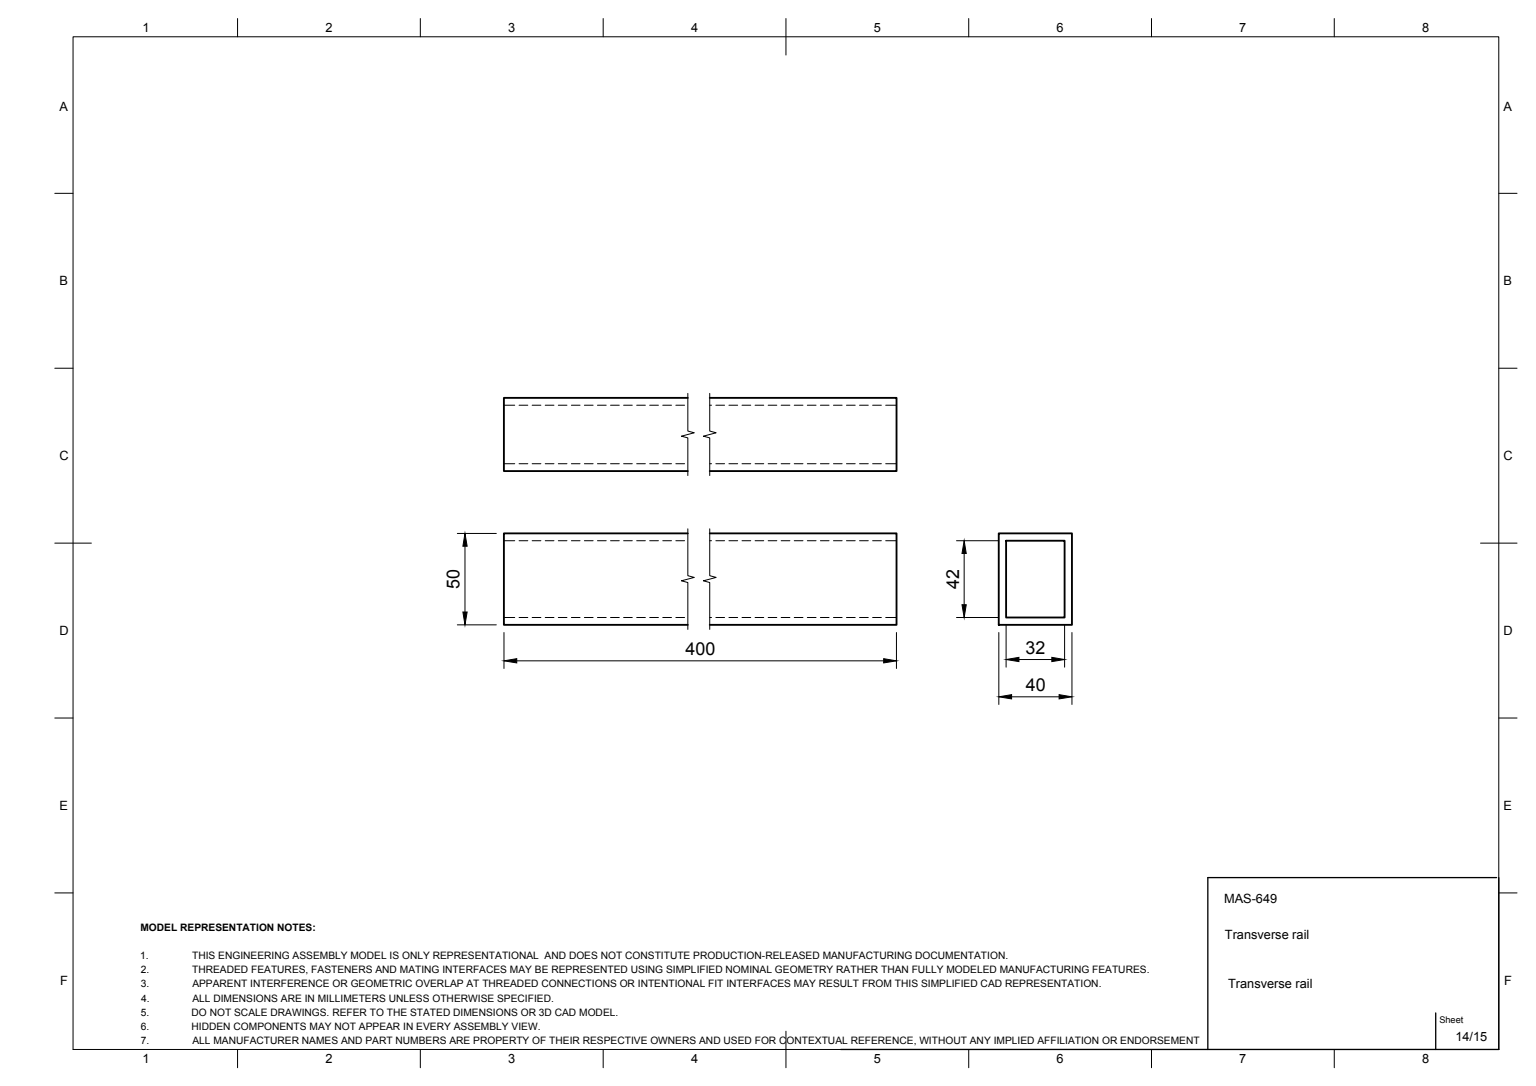
ISO-10303-21;
HEADER;
/* Generated by software containing ST-Developer
 * from STEP Tools, Inc. (www.steptools.com) 
 */

FILE_DESCRIPTION(
/* description */ ('Independent equipment support assembly with bolted 600 x 500 mm welde
d perimeter frame, four adjustable legs and swivel feet. Nominal overa
ll height 518 mm. No load rating assigned.'),
/* implementation_level */ '2;1');

FILE_NAME(
/* name */ 'Transverse rail.step',
/* time_stamp */ '2026-11-07T17:30:39-08:00',
/* author */ (''),
/* organization */ (''),
/* preprocessor_version */ 'ST-DEVELOPER v20.2',
/* originating_system */ 'Autodesk Translation Framework v15.17.0.0',
/* authorisation */ '');

FILE_SCHEMA (('AUTOMOTIVE_DESIGN { 1 0 10303 214 3 1 1 }'));
ENDSEC;

DATA;
#10=MECHANICAL_DESIGN_GEOMETRIC_PRESENTATION_REPRESENTATION('',(#2209),#63755);
#2177=SHAPE_REPRESENTATION_RELATIONSHIP('SRR','None',#63861,#2193);
#2193=ADVANCED_BREP_SHAPE_REPRESENTATION('',(#2225),#63739);
#2209=STYLED_ITEM('',(#63958),#2225);
#2225=MANIFOLD_SOLID_BREP('Body1',#14310);
#2242=FACE_BOUND('',#3084,.T.);
#2243=FACE_BOUND('',#3086,.T.);
#2313=FACE_OUTER_BOUND('',#3075,.T.);
#2314=FACE_OUTER_BOUND('',#3076,.T.);
#2315=FACE_OUTER_BOUND('',#3077,.T.);
#2316=FACE_OUTER_BOUND('',#3078,.T.);
#2317=FACE_OUTER_BOUND('',#3079,.T.);
#2318=FACE_OUTER_BOUND('',#3080,.T.);
#2319=FACE_OUTER_BOUND('',#3081,.T.);
#2320=FACE_OUTER_BOUND('',#3082,.T.);
#2321=FACE_OUTER_BOUND('',#3083,.T.);
#2322=FACE_OUTER_BOUND('',#3085,.T.);
#3075=EDGE_LOOP('',(#9175,#9176,#9177,#9178));
#3076=EDGE_LOOP('',(#9179,#9180,#9181,#9182));
#3077=EDGE_LOOP('',(#9183,#9184,#9185,#9186));
#3078=EDGE_LOOP('',(#9187,#9188,#9189,#9190));
#3079=EDGE_LOOP('',(#9191,#9192,#9193,#9194));
#3080=EDGE_LOOP('',(#9195,#9196,#9197,#9198));
#3081=EDGE_LOOP('',(#9199,#9200,#9201,#9202));
#3082=EDGE_LOOP('',(#9203,#9204,#9205,#9206));
#3083=EDGE_LOOP('',(#9207,#9208,#9209,#9210));
#3084=EDGE_LOOP('',(#9211,#9212,#9213,#9214));
#3085=EDGE_LOOP('',(#9215,#9216,#9217,#9218));
#3086=EDGE_LOOP('',(#9219,#9220,#9221,#9222));
#3910=LINE('',#18434,#4746);
#3911=LINE('',#18436,#4747);
#3912=LINE('',#18438,#4748);
#3913=LINE('',#18439,#4749);
#3914=LINE('',#18442,#4750);
#3915=LINE('',#18444,#4751);
#3916=LINE('',#18445,#4752);
#3917=LINE('',#18448,#4753);
#3918=LINE('',#18450,#4754);
#3919=LINE('',#18451,#4755);
#3920=LINE('',#18453,#4756);
#3921=LINE('',#18454,#4757);
#3922=LINE('',#18458,#4758);
#3923=LINE('',#18460,#4759);
#3924=LINE('',#18462,#4760);
#3925=LINE('',#18463,#4761);
#3926=LINE('',#18466,#4762);
#3927=LINE('',#18468,#4763);
#3928=LINE('',#18469,#4764);
#3929=LINE('',#18472,#4765);
#3930=LINE('',#18474,#4766);
#3931=LINE('',#18475,#4767);
#3932=LINE('',#18477,#4768);
#3933=LINE('',#18478,#4769);
#4746=VECTOR('',#15569,10.);
#4747=VECTOR('',#15570,10.);
#4748=VECTOR('',#15571,10.);
#4749=VECTOR('',#15572,10.);
#4750=VECTOR('',#15575,10.);
#4751=VECTOR('',#15576,10.);
#4752=VECTOR('',#15577,10.);
#4753=VECTOR('',#15580,10.);
#4754=VECTOR('',#15581,10.);
#4755=VECTOR('',#15582,10.);
#4756=VECTOR('',#15585,10.);
#4757=VECTOR('',#15586,10.);
#4758=VECTOR('',#15589,10.);
#4759=VECTOR('',#15590,10.);
#4760=VECTOR('',#15591,10.);
#4761=VECTOR('',#15592,10.);
#4762=VECTOR('',#15595,10.);
#4763=VECTOR('',#15596,10.);
#4764=VECTOR('',#15597,10.);
#4765=VECTOR('',#15600,10.);
#4766=VECTOR('',#15601,10.);
#4767=VECTOR('',#15602,10.);
#4768=VECTOR('',#15605,10.);
#4769=VECTOR('',#15606,10.);
#5574=VERTEX_POINT('',#18432);
#5575=VERTEX_POINT('',#18433);
#5576=VERTEX_POINT('',#18435);
#5577=VERTEX_POINT('',#18437);
#5578=VERTEX_POINT('',#18441);
#5579=VERTEX_POINT('',#18443);
#5580=VERTEX_POINT('',#18447);
#5581=VERTEX_POINT('',#18449);
#5582=VERTEX_POINT('',#18456);
#5583=VERTEX_POINT('',#18457);
#5584=VERTEX_POINT('',#18459);
#5585=VERTEX_POINT('',#18461);
#5586=VERTEX_POINT('',#18465);
#5587=VERTEX_POINT('',#18467);
#5588=VERTEX_POINT('',#18471);
#5589=VERTEX_POINT('',#18473);
#7010=EDGE_CURVE('',#5574,#5575,#3910,.T.);
#7011=EDGE_CURVE('',#5575,#5576,#3911,.T.);
#7012=EDGE_CURVE('',#5577,#5576,#3912,.T.);
#7013=EDGE_CURVE('',#5574,#5577,#3913,.T.);
#7014=EDGE_CURVE('',#5578,#5574,#3914,.T.);
#7015=EDGE_CURVE('',#5579,#5577,#3915,.T.);
#7016=EDGE_CURVE('',#5578,#5579,#3916,.T.);
#7017=EDGE_CURVE('',#5580,#5578,#3917,.T.);
#7018=EDGE_CURVE('',#5581,#5579,#3918,.T.);
#7019=EDGE_CURVE('',#5580,#5581,#3919,.T.);
#7020=EDGE_CURVE('',#5575,#5580,#3920,.T.);
#7021=EDGE_CURVE('',#5576,#5581,#3921,.T.);
#7022=EDGE_CURVE('',#5582,#5583,#3922,.T.);
#7023=EDGE_CURVE('',#5583,#5584,#3923,.T.);
#7024=EDGE_CURVE('',#5585,#5584,#3924,.T.);
#7025=EDGE_CURVE('',#5582,#5585,#3925,.T.);
#7026=EDGE_CURVE('',#5586,#5582,#3926,.T.);
#7027=EDGE_CURVE('',#5587,#5585,#3927,.T.);
#7028=EDGE_CURVE('',#5586,#5587,#3928,.T.);
#7029=EDGE_CURVE('',#5588,#5586,#3929,.T.);
#7030=EDGE_CURVE('',#5589,#5587,#3930,.T.);
#7031=EDGE_CURVE('',#5588,#5589,#3931,.T.);
#7032=EDGE_CURVE('',#5583,#5588,#3932,.T.);
#7033=EDGE_CURVE('',#5584,#5589,#3933,.T.);
#9175=ORIENTED_EDGE('',*,*,#7010,.T.);
#9176=ORIENTED_EDGE('',*,*,#7011,.T.);
#9177=ORIENTED_EDGE('',*,*,#7012,.F.);
#9178=ORIENTED_EDGE('',*,*,#7013,.F.);
#9179=ORIENTED_EDGE('',*,*,#7014,.T.);
#9180=ORIENTED_EDGE('',*,*,#7013,.T.);
#9181=ORIENTED_EDGE('',*,*,#7015,.F.);
#9182=ORIENTED_EDGE('',*,*,#7016,.F.);
#9183=ORIENTED_EDGE('',*,*,#7017,.T.);
#9184=ORIENTED_EDGE('',*,*,#7016,.T.);
#9185=ORIENTED_EDGE('',*,*,#7018,.F.);
#9186=ORIENTED_EDGE('',*,*,#7019,.F.);
#9187=ORIENTED_EDGE('',*,*,#7020,.T.);
#9188=ORIENTED_EDGE('',*,*,#7019,.T.);
#9189=ORIENTED_EDGE('',*,*,#7021,.F.);
#9190=ORIENTED_EDGE('',*,*,#7011,.F.);
#9191=ORIENTED_EDGE('',*,*,#7022,.T.);
#9192=ORIENTED_EDGE('',*,*,#7023,.T.);
#9193=ORIENTED_EDGE('',*,*,#7024,.F.);
#9194=ORIENTED_EDGE('',*,*,#7025,.F.);
#9195=ORIENTED_EDGE('',*,*,#7026,.T.);
#9196=ORIENTED_EDGE('',*,*,#7025,.T.);
#9197=ORIENTED_EDGE('',*,*,#7027,.F.);
#9198=ORIENTED_EDGE('',*,*,#7028,.F.);
#9199=ORIENTED_EDGE('',*,*,#7029,.T.);
#9200=ORIENTED_EDGE('',*,*,#7028,.T.);
#9201=ORIENTED_EDGE('',*,*,#7030,.F.);
#9202=ORIENTED_EDGE('',*,*,#7031,.F.);
#9203=ORIENTED_EDGE('',*,*,#7032,.T.);
#9204=ORIENTED_EDGE('',*,*,#7031,.T.);
#9205=ORIENTED_EDGE('',*,*,#7033,.F.);
#9206=ORIENTED_EDGE('',*,*,#7023,.F.);
#9207=ORIENTED_EDGE('',*,*,#7033,.T.);
#9208=ORIENTED_EDGE('',*,*,#7030,.T.);
#9209=ORIENTED_EDGE('',*,*,#7027,.T.);
#9210=ORIENTED_EDGE('',*,*,#7024,.T.);
#9211=ORIENTED_EDGE('',*,*,#7021,.T.);
#9212=ORIENTED_EDGE('',*,*,#7018,.T.);
#9213=ORIENTED_EDGE('',*,*,#7015,.T.);
#9214=ORIENTED_EDGE('',*,*,#7012,.T.);
#9215=ORIENTED_EDGE('',*,*,#7032,.F.);
#9216=ORIENTED_EDGE('',*,*,#7022,.F.);
#9217=ORIENTED_EDGE('',*,*,#7026,.F.);
#9218=ORIENTED_EDGE('',*,*,#7029,.F.);
#9219=ORIENTED_EDGE('',*,*,#7020,.F.);
#9220=ORIENTED_EDGE('',*,*,#7010,.F.);
#9221=ORIENTED_EDGE('',*,*,#7014,.F.);
#9222=ORIENTED_EDGE('',*,*,#7017,.F.);
#13419=PLANE('',#14516);
#13420=PLANE('',#14517);
#13421=PLANE('',#14518);
#13422=PLANE('',#14519);
#13423=PLANE('',#14520);
#13424=PLANE('',#14521);
#13425=PLANE('',#14522);
#13426=PLANE('',#14523);
#13427=PLANE('',#14524);
#13428=PLANE('',#14525);
#13559=ADVANCED_FACE('',(#2313),#13419,.T.);
#13560=ADVANCED_FACE('',(#2314),#13420,.T.);
#13561=ADVANCED_FACE('',(#2315),#13421,.T.);
#13562=ADVANCED_FACE('',(#2316),#13422,.T.);
#13563=ADVANCED_FACE('',(#2317),#13423,.T.);
#13564=ADVANCED_FACE('',(#2318),#13424,.T.);
#13565=ADVANCED_FACE('',(#2319),#13425,.T.);
#13566=ADVANCED_FACE('',(#2320),#13426,.T.);
#13567=ADVANCED_FACE('',(#2321,#2242),#13427,.T.);
#13568=ADVANCED_FACE('',(#2322,#2243),#13428,.F.);
#14310=CLOSED_SHELL('',(#13559,#13560,#13561,#13562,#13563,#13564,#13565,
#13566,#13567,#13568));
#14515=AXIS2_PLACEMENT_3D('',#18430,#15565,#15566);
#14516=AXIS2_PLACEMENT_3D('',#18431,#15567,#15568);
#14517=AXIS2_PLACEMENT_3D('',#18440,#15573,#15574);
#14518=AXIS2_PLACEMENT_3D('',#18446,#15578,#15579);
#14519=AXIS2_PLACEMENT_3D('',#18452,#15583,#15584);
#14520=AXIS2_PLACEMENT_3D('',#18455,#15587,#15588);
#14521=AXIS2_PLACEMENT_3D('',#18464,#15593,#15594);
#14522=AXIS2_PLACEMENT_3D('',#18470,#15598,#15599);
#14523=AXIS2_PLACEMENT_3D('',#18476,#15603,#15604);
#14524=AXIS2_PLACEMENT_3D('',#18479,#15607,#15608);
#14525=AXIS2_PLACEMENT_3D('',#18480,#15609,#15610);
#15565=DIRECTION('axis',(0.,0.,1.));
#15566=DIRECTION('refdir',(1.,0.,0.));
#15567=DIRECTION('center_axis',(0.,1.,0.));
#15568=DIRECTION('ref_axis',(-1.,0.,0.));
#15569=DIRECTION('',(-1.,0.,0.));
#15570=DIRECTION('',(0.,0.,1.));
#15571=DIRECTION('',(-1.,0.,0.));
#15572=DIRECTION('',(0.,0.,1.));
#15573=DIRECTION('center_axis',(-1.,0.,0.));
#15574=DIRECTION('ref_axis',(0.,-1.,0.));
#15575=DIRECTION('',(0.,-1.,0.));
#15576=DIRECTION('',(0.,-1.,0.));
#15577=DIRECTION('',(0.,0.,1.));
#15578=DIRECTION('center_axis',(0.,-1.,0.));
#15579=DIRECTION('ref_axis',(1.,0.,0.));
#15580=DIRECTION('',(1.,0.,0.));
#15581=DIRECTION('',(1.,0.,0.));
#15582=DIRECTION('',(0.,0.,1.));
#15583=DIRECTION('center_axis',(1.,0.,0.));
#15584=DIRECTION('ref_axis',(0.,1.,0.));
#15585=DIRECTION('',(0.,1.,0.));
#15586=DIRECTION('',(0.,1.,0.));
#15587=DIRECTION('center_axis',(0.,1.,0.));
#15588=DIRECTION('ref_axis',(-1.,0.,0.));
#15589=DIRECTION('',(-1.,0.,0.));
#15590=DIRECTION('',(0.,0.,1.));
#15591=DIRECTION('',(-1.,0.,0.));
#15592=DIRECTION('',(0.,0.,1.));
#15593=DIRECTION('center_axis',(1.,0.,0.));
#15594=DIRECTION('ref_axis',(0.,1.,0.));
#15595=DIRECTION('',(0.,1.,0.));
#15596=DIRECTION('',(0.,1.,0.));
#15597=DIRECTION('',(0.,0.,1.));
#15598=DIRECTION('center_axis',(0.,-1.,0.));
#15599=DIRECTION('ref_axis',(1.,0.,0.));
#15600=DIRECTION('',(1.,0.,0.));
#15601=DIRECTION('',(1.,0.,0.));
#15602=DIRECTION('',(0.,0.,1.));
#15603=DIRECTION('center_axis',(-1.,0.,0.));
#15604=DIRECTION('ref_axis',(0.,-1.,0.));
#15605=DIRECTION('',(0.,-1.,0.));
#15606=DIRECTION('',(0.,-1.,0.));
#15607=DIRECTION('center_axis',(0.,0.,1.));
#15608=DIRECTION('ref_axis',(1.,0.,0.));
#15609=DIRECTION('center_axis',(0.,0.,1.));
#15610=DIRECTION('ref_axis',(1.,0.,0.));
#18430=CARTESIAN_POINT('',(0.,0.,0.));
#18431=CARTESIAN_POINT('Origin',(16.,-21.,0.));
#18432=CARTESIAN_POINT('',(16.,-21.,0.));
#18433=CARTESIAN_POINT('',(-16.,-21.,0.));
#18434=CARTESIAN_POINT('',(-16.,-21.,0.));
#18435=CARTESIAN_POINT('',(-16.,-21.,400.));
#18436=CARTESIAN_POINT('',(-16.,-21.,0.));
#18437=CARTESIAN_POINT('',(16.,-21.,400.));
#18438=CARTESIAN_POINT('',(-16.,-21.,400.));
#18439=CARTESIAN_POINT('',(16.,-21.,0.));
#18440=CARTESIAN_POINT('Origin',(16.,21.,0.));
#18441=CARTESIAN_POINT('',(16.,21.,0.));
#18442=CARTESIAN_POINT('',(16.,-21.,0.));
#18443=CARTESIAN_POINT('',(16.,21.,400.));
#18444=CARTESIAN_POINT('',(16.,-21.,400.));
#18445=CARTESIAN_POINT('',(16.,21.,0.));
#18446=CARTESIAN_POINT('Origin',(-16.,21.,0.));
#18447=CARTESIAN_POINT('',(-16.,21.,0.));
#18448=CARTESIAN_POINT('',(16.,21.,0.));
#18449=CARTESIAN_POINT('',(-16.,21.,400.));
#18450=CARTESIAN_POINT('',(16.,21.,400.));
#18451=CARTESIAN_POINT('',(-16.,21.,0.));
#18452=CARTESIAN_POINT('Origin',(-16.,-21.,0.));
#18453=CARTESIAN_POINT('',(-16.,21.,0.));
#18454=CARTESIAN_POINT('',(-16.,21.,400.));
#18455=CARTESIAN_POINT('Origin',(20.,25.,0.));
#18456=CARTESIAN_POINT('',(20.,25.,0.));
#18457=CARTESIAN_POINT('',(-20.,25.,0.));
#18458=CARTESIAN_POINT('',(20.,25.,0.));
#18459=CARTESIAN_POINT('',(-20.,25.,400.));
#18460=CARTESIAN_POINT('',(-20.,25.,0.));
#18461=CARTESIAN_POINT('',(20.,25.,400.));
#18462=CARTESIAN_POINT('',(20.,25.,400.));
#18463=CARTESIAN_POINT('',(20.,25.,0.));
#18464=CARTESIAN_POINT('Origin',(20.,-25.,0.));
#18465=CARTESIAN_POINT('',(20.,-25.,0.));
#18466=CARTESIAN_POINT('',(20.,-25.,0.));
#18467=CARTESIAN_POINT('',(20.,-25.,400.));
#18468=CARTESIAN_POINT('',(20.,-25.,400.));
#18469=CARTESIAN_POINT('',(20.,-25.,0.));
#18470=CARTESIAN_POINT('Origin',(-20.,-25.,0.));
#18471=CARTESIAN_POINT('',(-20.,-25.,0.));
#18472=CARTESIAN_POINT('',(-20.,-25.,0.));
#18473=CARTESIAN_POINT('',(-20.,-25.,400.));
#18474=CARTESIAN_POINT('',(-20.,-25.,400.));
#18475=CARTESIAN_POINT('',(-20.,-25.,0.));
#18476=CARTESIAN_POINT('Origin',(-20.,25.,0.));
#18477=CARTESIAN_POINT('',(-20.,25.,0.));
#18478=CARTESIAN_POINT('',(-20.,25.,400.));
#18479=CARTESIAN_POINT('Origin',(0.,0.,400.));
#18480=CARTESIAN_POINT('Origin',(0.,0.,0.));
#63719=UNCERTAINTY_MEASURE_WITH_UNIT(LENGTH_MEASURE(0.01),#63756,
'DISTANCE_ACCURACY_VALUE',
'Maximum model space distance between geometric entities at asserted c
onnectivities');
#63735=UNCERTAINTY_MEASURE_WITH_UNIT(LENGTH_MEASURE(0.01),#63756,
'DISTANCE_ACCURACY_VALUE',
'Maximum model space distance between geometric entities at asserted c
onnectivities');
#63739=(
GEOMETRIC_REPRESENTATION_CONTEXT(3)
GLOBAL_UNCERTAINTY_ASSIGNED_CONTEXT((#63719))
GLOBAL_UNIT_ASSIGNED_CONTEXT((#63756,#63758,#63759))
REPRESENTATION_CONTEXT('','3D')
);
#63755=(
GEOMETRIC_REPRESENTATION_CONTEXT(3)
GLOBAL_UNCERTAINTY_ASSIGNED_CONTEXT((#63735))
GLOBAL_UNIT_ASSIGNED_CONTEXT((#63756,#63758,#63759))
REPRESENTATION_CONTEXT('','3D')
);
#63756=(
LENGTH_UNIT()
NAMED_UNIT(*)
SI_UNIT(.MILLI.,.METRE.)
);
#63758=(
NAMED_UNIT(*)
PLANE_ANGLE_UNIT()
SI_UNIT($,.RADIAN.)
);
#63759=(
NAMED_UNIT(*)
SI_UNIT($,.STERADIAN.)
SOLID_ANGLE_UNIT()
);
#63763=SHAPE_DEFINITION_REPRESENTATION(#63782,#63861);
#63782=PRODUCT_DEFINITION_SHAPE('',$,#63881);
#63861=SHAPE_REPRESENTATION('',(#14515),#63739);
#63877=PRODUCT_DEFINITION_CONTEXT('part definition',#63936,'design');
#63881=PRODUCT_DEFINITION('Transverse rail','Transverse rail',#63900,#63877);
#63900=PRODUCT_DEFINITION_FORMATION('',$,#63941);
#63936=APPLICATION_CONTEXT(
'Core Data for Automotive Mechanical Design Process');
#63937=PRODUCT_CONTEXT('part definition',#63936,'mechanical');
#63941=PRODUCT('Transverse rail','Transverse rail',
'Steel rectangular hollow section, 50 x 40 mm, 4 mm wall. Square cut e
nds; weld to adjoining rails and corner plates.',(#63937));
#63958=PRESENTATION_STYLE_ASSIGNMENT((#63965));
#63965=SURFACE_STYLE_USAGE(.BOTH.,#63972);
#63972=SURFACE_SIDE_STYLE('',(#63979));
#63979=SURFACE_STYLE_FILL_AREA(#63986);
#63986=FILL_AREA_STYLE('Dark blue',(#63993));
#63993=FILL_AREA_STYLE_COLOUR('Dark blue',#64000);
#64000=COLOUR_RGB('Dark blue',0.0901960784313725,0.270588235294118,0.513725490196078);
ENDSEC;
END-ISO-10303-21;
